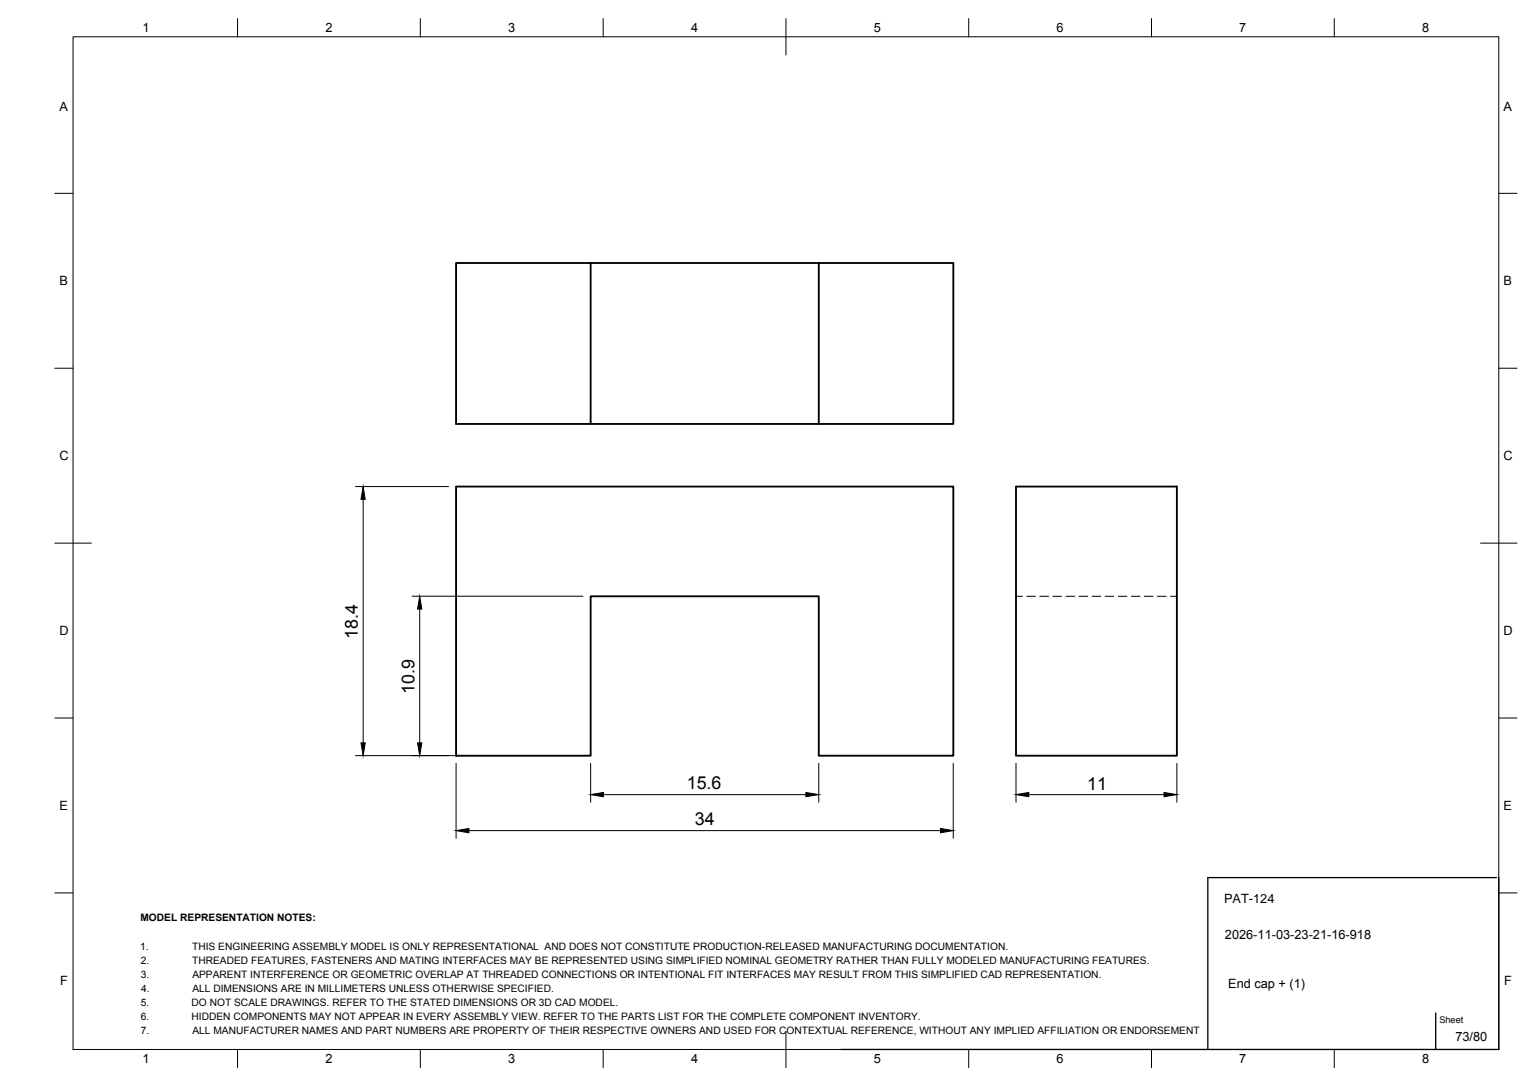
ISO-10303-21;
HEADER;
/* Generated by software containing ST-Developer
 * from STEP Tools, Inc. (www.steptools.com) 
 */

FILE_DESCRIPTION(
/* description */ ('XY cross-slide table'),
/* implementation_level */ '2;1');

FILE_NAME(
/* name */ 'End cap + (1).step',
/* time_stamp */ '2026-10-28T03:22:46-07:00',
/* author */ (''),
/* organization */ (''),
/* preprocessor_version */ 'ST-DEVELOPER v20.2',
/* originating_system */ 'Autodesk Translation Framework v15.17.0.0',
/* authorisation */ '');

FILE_SCHEMA (('AUTOMOTIVE_DESIGN { 1 0 10303 214 3 1 1 }'));
ENDSEC;

DATA;
#10=MECHANICAL_DESIGN_GEOMETRIC_PRESENTATION_REPRESENTATION('',(#1766),#62984);
#1570=SHAPE_REPRESENTATION_RELATIONSHIP('SRR','None',#63429,#1653);
#1653=ADVANCED_BREP_SHAPE_REPRESENTATION('',(#1874),#62966);
#1766=STYLED_ITEM('',(#63905),#1874);
#1874=MANIFOLD_SOLID_BREP('Body1',#23065);
#2749=PLANE('',#25946);
#2750=PLANE('',#25947);
#2751=PLANE('',#25948);
#2752=PLANE('',#25949);
#2753=PLANE('',#25950);
#2754=PLANE('',#25951);
#2755=PLANE('',#25952);
#2756=PLANE('',#25953);
#2757=PLANE('',#25954);
#2758=PLANE('',#25955);
#3857=FACE_OUTER_BOUND('',#5541,.T.);
#3858=FACE_OUTER_BOUND('',#5542,.T.);
#3859=FACE_OUTER_BOUND('',#5543,.T.);
#3860=FACE_OUTER_BOUND('',#5544,.T.);
#3861=FACE_OUTER_BOUND('',#5545,.T.);
#3862=FACE_OUTER_BOUND('',#5546,.T.);
#3863=FACE_OUTER_BOUND('',#5547,.T.);
#3864=FACE_OUTER_BOUND('',#5548,.T.);
#3865=FACE_OUTER_BOUND('',#5549,.T.);
#3866=FACE_OUTER_BOUND('',#5550,.T.);
#5541=EDGE_LOOP('',(#19434,#19435,#19436,#19437));
#5542=EDGE_LOOP('',(#19438,#19439,#19440,#19441));
#5543=EDGE_LOOP('',(#19442,#19443,#19444,#19445));
#5544=EDGE_LOOP('',(#19446,#19447,#19448,#19449));
#5545=EDGE_LOOP('',(#19450,#19451,#19452,#19453));
#5546=EDGE_LOOP('',(#19454,#19455,#19456,#19457));
#5547=EDGE_LOOP('',(#19458,#19459,#19460,#19461));
#5548=EDGE_LOOP('',(#19462,#19463,#19464,#19465));
#5549=EDGE_LOOP('',(#19466,#19467,#19468,#19469,#19470,#19471,#19472,#19473));
#5550=EDGE_LOOP('',(#19474,#19475,#19476,#19477,#19478,#19479,#19480,#19481));
#7004=LINE('',#50067,#8491);
#7005=LINE('',#50069,#8492);
#7006=LINE('',#50071,#8493);
#7007=LINE('',#50072,#8494);
#7008=LINE('',#50075,#8495);
#7009=LINE('',#50077,#8496);
#7010=LINE('',#50078,#8497);
#7011=LINE('',#50081,#8498);
#7012=LINE('',#50083,#8499);
#7013=LINE('',#50084,#8500);
#7014=LINE('',#50087,#8501);
#7015=LINE('',#50089,#8502);
#7016=LINE('',#50090,#8503);
#7017=LINE('',#50093,#8504);
#7018=LINE('',#50095,#8505);
#7019=LINE('',#50096,#8506);
#7020=LINE('',#50099,#8507);
#7021=LINE('',#50101,#8508);
#7022=LINE('',#50102,#8509);
#7023=LINE('',#50105,#8510);
#7024=LINE('',#50107,#8511);
#7025=LINE('',#50108,#8512);
#7026=LINE('',#50110,#8513);
#7027=LINE('',#50111,#8514);
#8491=VECTOR('',#31453,1.);
#8492=VECTOR('',#31454,1.);
#8493=VECTOR('',#31455,1.);
#8494=VECTOR('',#31456,1.);
#8495=VECTOR('',#31459,1.);
#8496=VECTOR('',#31460,1.);
#8497=VECTOR('',#31461,1.);
#8498=VECTOR('',#31464,1.);
#8499=VECTOR('',#31465,1.);
#8500=VECTOR('',#31466,1.);
#8501=VECTOR('',#31469,1.);
#8502=VECTOR('',#31470,1.);
#8503=VECTOR('',#31471,1.);
#8504=VECTOR('',#31474,1.);
#8505=VECTOR('',#31475,1.);
#8506=VECTOR('',#31476,1.);
#8507=VECTOR('',#31479,1.);
#8508=VECTOR('',#31480,1.);
#8509=VECTOR('',#31481,1.);
#8510=VECTOR('',#31484,1.);
#8511=VECTOR('',#31485,1.);
#8512=VECTOR('',#31486,1.);
#8513=VECTOR('',#31489,1.);
#8514=VECTOR('',#31490,1.);
#11306=VERTEX_POINT('',#50065);
#11307=VERTEX_POINT('',#50066);
#11308=VERTEX_POINT('',#50068);
#11309=VERTEX_POINT('',#50070);
#11310=VERTEX_POINT('',#50074);
#11311=VERTEX_POINT('',#50076);
#11312=VERTEX_POINT('',#50080);
#11313=VERTEX_POINT('',#50082);
#11314=VERTEX_POINT('',#50086);
#11315=VERTEX_POINT('',#50088);
#11316=VERTEX_POINT('',#50092);
#11317=VERTEX_POINT('',#50094);
#11318=VERTEX_POINT('',#50098);
#11319=VERTEX_POINT('',#50100);
#11320=VERTEX_POINT('',#50104);
#11321=VERTEX_POINT('',#50106);
#14101=EDGE_CURVE('',#11306,#11307,#7004,.T.);
#14102=EDGE_CURVE('',#11307,#11308,#7005,.T.);
#14103=EDGE_CURVE('',#11309,#11308,#7006,.T.);
#14104=EDGE_CURVE('',#11306,#11309,#7007,.T.);
#14105=EDGE_CURVE('',#11310,#11306,#7008,.T.);
#14106=EDGE_CURVE('',#11311,#11309,#7009,.T.);
#14107=EDGE_CURVE('',#11310,#11311,#7010,.T.);
#14108=EDGE_CURVE('',#11312,#11310,#7011,.T.);
#14109=EDGE_CURVE('',#11313,#11311,#7012,.T.);
#14110=EDGE_CURVE('',#11312,#11313,#7013,.T.);
#14111=EDGE_CURVE('',#11314,#11312,#7014,.T.);
#14112=EDGE_CURVE('',#11315,#11313,#7015,.T.);
#14113=EDGE_CURVE('',#11314,#11315,#7016,.T.);
#14114=EDGE_CURVE('',#11316,#11314,#7017,.T.);
#14115=EDGE_CURVE('',#11317,#11315,#7018,.T.);
#14116=EDGE_CURVE('',#11316,#11317,#7019,.T.);
#14117=EDGE_CURVE('',#11318,#11316,#7020,.T.);
#14118=EDGE_CURVE('',#11319,#11317,#7021,.T.);
#14119=EDGE_CURVE('',#11318,#11319,#7022,.T.);
#14120=EDGE_CURVE('',#11320,#11318,#7023,.T.);
#14121=EDGE_CURVE('',#11321,#11319,#7024,.T.);
#14122=EDGE_CURVE('',#11320,#11321,#7025,.T.);
#14123=EDGE_CURVE('',#11307,#11320,#7026,.T.);
#14124=EDGE_CURVE('',#11308,#11321,#7027,.T.);
#19434=ORIENTED_EDGE('',*,*,#14101,.T.);
#19435=ORIENTED_EDGE('',*,*,#14102,.T.);
#19436=ORIENTED_EDGE('',*,*,#14103,.F.);
#19437=ORIENTED_EDGE('',*,*,#14104,.F.);
#19438=ORIENTED_EDGE('',*,*,#14105,.T.);
#19439=ORIENTED_EDGE('',*,*,#14104,.T.);
#19440=ORIENTED_EDGE('',*,*,#14106,.F.);
#19441=ORIENTED_EDGE('',*,*,#14107,.F.);
#19442=ORIENTED_EDGE('',*,*,#14108,.T.);
#19443=ORIENTED_EDGE('',*,*,#14107,.T.);
#19444=ORIENTED_EDGE('',*,*,#14109,.F.);
#19445=ORIENTED_EDGE('',*,*,#14110,.F.);
#19446=ORIENTED_EDGE('',*,*,#14111,.T.);
#19447=ORIENTED_EDGE('',*,*,#14110,.T.);
#19448=ORIENTED_EDGE('',*,*,#14112,.F.);
#19449=ORIENTED_EDGE('',*,*,#14113,.F.);
#19450=ORIENTED_EDGE('',*,*,#14114,.T.);
#19451=ORIENTED_EDGE('',*,*,#14113,.T.);
#19452=ORIENTED_EDGE('',*,*,#14115,.F.);
#19453=ORIENTED_EDGE('',*,*,#14116,.F.);
#19454=ORIENTED_EDGE('',*,*,#14117,.T.);
#19455=ORIENTED_EDGE('',*,*,#14116,.T.);
#19456=ORIENTED_EDGE('',*,*,#14118,.F.);
#19457=ORIENTED_EDGE('',*,*,#14119,.F.);
#19458=ORIENTED_EDGE('',*,*,#14120,.T.);
#19459=ORIENTED_EDGE('',*,*,#14119,.T.);
#19460=ORIENTED_EDGE('',*,*,#14121,.F.);
#19461=ORIENTED_EDGE('',*,*,#14122,.F.);
#19462=ORIENTED_EDGE('',*,*,#14123,.T.);
#19463=ORIENTED_EDGE('',*,*,#14122,.T.);
#19464=ORIENTED_EDGE('',*,*,#14124,.F.);
#19465=ORIENTED_EDGE('',*,*,#14102,.F.);
#19466=ORIENTED_EDGE('',*,*,#14124,.T.);
#19467=ORIENTED_EDGE('',*,*,#14121,.T.);
#19468=ORIENTED_EDGE('',*,*,#14118,.T.);
#19469=ORIENTED_EDGE('',*,*,#14115,.T.);
#19470=ORIENTED_EDGE('',*,*,#14112,.T.);
#19471=ORIENTED_EDGE('',*,*,#14109,.T.);
#19472=ORIENTED_EDGE('',*,*,#14106,.T.);
#19473=ORIENTED_EDGE('',*,*,#14103,.T.);
#19474=ORIENTED_EDGE('',*,*,#14123,.F.);
#19475=ORIENTED_EDGE('',*,*,#14101,.F.);
#19476=ORIENTED_EDGE('',*,*,#14105,.F.);
#19477=ORIENTED_EDGE('',*,*,#14108,.F.);
#19478=ORIENTED_EDGE('',*,*,#14111,.F.);
#19479=ORIENTED_EDGE('',*,*,#14114,.F.);
#19480=ORIENTED_EDGE('',*,*,#14117,.F.);
#19481=ORIENTED_EDGE('',*,*,#14120,.F.);
#22638=ADVANCED_FACE('',(#3857),#2749,.T.);
#22639=ADVANCED_FACE('',(#3858),#2750,.T.);
#22640=ADVANCED_FACE('',(#3859),#2751,.T.);
#22641=ADVANCED_FACE('',(#3860),#2752,.T.);
#22642=ADVANCED_FACE('',(#3861),#2753,.T.);
#22643=ADVANCED_FACE('',(#3862),#2754,.T.);
#22644=ADVANCED_FACE('',(#3863),#2755,.T.);
#22645=ADVANCED_FACE('',(#3864),#2756,.T.);
#22646=ADVANCED_FACE('',(#3865),#2757,.T.);
#22647=ADVANCED_FACE('',(#3866),#2758,.F.);
#23065=CLOSED_SHELL('',(#22638,#22639,#22640,#22641,#22642,#22643,#22644,
#22645,#22646,#22647));
#25945=AXIS2_PLACEMENT_3D('',#50063,#31449,#31450);
#25946=AXIS2_PLACEMENT_3D('',#50064,#31451,#31452);
#25947=AXIS2_PLACEMENT_3D('',#50073,#31457,#31458);
#25948=AXIS2_PLACEMENT_3D('',#50079,#31462,#31463);
#25949=AXIS2_PLACEMENT_3D('',#50085,#31467,#31468);
#25950=AXIS2_PLACEMENT_3D('',#50091,#31472,#31473);
#25951=AXIS2_PLACEMENT_3D('',#50097,#31477,#31478);
#25952=AXIS2_PLACEMENT_3D('',#50103,#31482,#31483);
#25953=AXIS2_PLACEMENT_3D('',#50109,#31487,#31488);
#25954=AXIS2_PLACEMENT_3D('',#50112,#31491,#31492);
#25955=AXIS2_PLACEMENT_3D('',#50113,#31493,#31494);
#31449=DIRECTION('axis',(0.,0.,1.));
#31450=DIRECTION('refdir',(1.,0.,0.));
#31451=DIRECTION('center_axis',(0.,0.,1.));
#31452=DIRECTION('ref_axis',(0.,-1.,0.));
#31453=DIRECTION('',(0.,-1.,0.));
#31454=DIRECTION('',(1.,0.,0.));
#31455=DIRECTION('',(0.,-1.,0.));
#31456=DIRECTION('',(1.,0.,0.));
#31457=DIRECTION('center_axis',(0.,1.,0.));
#31458=DIRECTION('ref_axis',(0.,0.,1.));
#31459=DIRECTION('',(0.,0.,1.));
#31460=DIRECTION('',(0.,0.,1.));
#31461=DIRECTION('',(1.,0.,0.));
#31462=DIRECTION('center_axis',(0.,0.,-1.));
#31463=DIRECTION('ref_axis',(0.,1.,0.));
#31464=DIRECTION('',(0.,1.,0.));
#31465=DIRECTION('',(0.,1.,0.));
#31466=DIRECTION('',(1.,0.,0.));
#31467=DIRECTION('center_axis',(0.,-1.,0.));
#31468=DIRECTION('ref_axis',(0.,0.,-1.));
#31469=DIRECTION('',(0.,0.,-1.));
#31470=DIRECTION('',(0.,0.,-1.));
#31471=DIRECTION('',(1.,0.,0.));
#31472=DIRECTION('center_axis',(0.,0.,-1.));
#31473=DIRECTION('ref_axis',(0.,1.,0.));
#31474=DIRECTION('',(0.,1.,0.));
#31475=DIRECTION('',(0.,1.,0.));
#31476=DIRECTION('',(1.,0.,0.));
#31477=DIRECTION('center_axis',(0.,1.,0.));
#31478=DIRECTION('ref_axis',(0.,0.,1.));
#31479=DIRECTION('',(0.,0.,1.));
#31480=DIRECTION('',(0.,0.,1.));
#31481=DIRECTION('',(1.,0.,0.));
#31482=DIRECTION('center_axis',(0.,0.,-1.));
#31483=DIRECTION('ref_axis',(0.,1.,0.));
#31484=DIRECTION('',(0.,1.,0.));
#31485=DIRECTION('',(0.,1.,0.));
#31486=DIRECTION('',(1.,0.,0.));
#31487=DIRECTION('center_axis',(0.,-1.,0.));
#31488=DIRECTION('ref_axis',(0.,0.,-1.));
#31489=DIRECTION('',(0.,0.,-1.));
#31490=DIRECTION('',(0.,0.,-1.));
#31491=DIRECTION('center_axis',(1.,0.,0.));
#31492=DIRECTION('ref_axis',(0.,0.,-1.));
#31493=DIRECTION('center_axis',(1.,0.,0.));
#31494=DIRECTION('ref_axis',(0.,0.,-1.));
#50063=CARTESIAN_POINT('',(0.,0.,0.));
#50064=CARTESIAN_POINT('Origin',(1.97,1.7,2.3));
#50065=CARTESIAN_POINT('',(1.97,1.7,2.3));
#50066=CARTESIAN_POINT('',(1.97,-1.7,2.3));
#50067=CARTESIAN_POINT('',(1.97,1.7,2.3));
#50068=CARTESIAN_POINT('',(3.07,-1.7,2.3));
#50069=CARTESIAN_POINT('',(1.97,-1.7,2.3));
#50070=CARTESIAN_POINT('',(3.07,1.7,2.3));
#50071=CARTESIAN_POINT('',(3.07,1.7,2.3));
#50072=CARTESIAN_POINT('',(1.97,1.7,2.3));
#50073=CARTESIAN_POINT('Origin',(1.97,1.7,0.46));
#50074=CARTESIAN_POINT('',(1.97,1.7,0.46));
#50075=CARTESIAN_POINT('',(1.97,1.7,0.46));
#50076=CARTESIAN_POINT('',(3.07,1.7,0.46));
#50077=CARTESIAN_POINT('',(3.07,1.7,0.46));
#50078=CARTESIAN_POINT('',(1.97,1.7,0.46));
#50079=CARTESIAN_POINT('Origin',(1.97,0.78,0.46));
#50080=CARTESIAN_POINT('',(1.97,0.78,0.46));
#50081=CARTESIAN_POINT('',(1.97,0.78,0.46));
#50082=CARTESIAN_POINT('',(3.07,0.78,0.46));
#50083=CARTESIAN_POINT('',(3.07,0.78,0.46));
#50084=CARTESIAN_POINT('',(1.97,0.78,0.46));
#50085=CARTESIAN_POINT('Origin',(1.97,0.78,1.55));
#50086=CARTESIAN_POINT('',(1.97,0.78,1.55));
#50087=CARTESIAN_POINT('',(1.97,0.78,1.55));
#50088=CARTESIAN_POINT('',(3.07,0.78,1.55));
#50089=CARTESIAN_POINT('',(3.07,0.78,1.55));
#50090=CARTESIAN_POINT('',(1.97,0.78,1.55));
#50091=CARTESIAN_POINT('Origin',(1.97,-0.78,1.55));
#50092=CARTESIAN_POINT('',(1.97,-0.78,1.55));
#50093=CARTESIAN_POINT('',(1.97,-0.78,1.55));
#50094=CARTESIAN_POINT('',(3.07,-0.78,1.55));
#50095=CARTESIAN_POINT('',(3.07,-0.78,1.55));
#50096=CARTESIAN_POINT('',(1.97,-0.78,1.55));
#50097=CARTESIAN_POINT('Origin',(1.97,-0.78,0.46));
#50098=CARTESIAN_POINT('',(1.97,-0.78,0.46));
#50099=CARTESIAN_POINT('',(1.97,-0.78,0.46));
#50100=CARTESIAN_POINT('',(3.07,-0.78,0.46));
#50101=CARTESIAN_POINT('',(3.07,-0.78,0.46));
#50102=CARTESIAN_POINT('',(1.97,-0.78,0.46));
#50103=CARTESIAN_POINT('Origin',(1.97,-1.7,0.46));
#50104=CARTESIAN_POINT('',(1.97,-1.7,0.46));
#50105=CARTESIAN_POINT('',(1.97,-1.7,0.46));
#50106=CARTESIAN_POINT('',(3.07,-1.7,0.46));
#50107=CARTESIAN_POINT('',(3.07,-1.7,0.46));
#50108=CARTESIAN_POINT('',(1.97,-1.7,0.46));
#50109=CARTESIAN_POINT('Origin',(1.97,-1.7,2.3));
#50110=CARTESIAN_POINT('',(1.97,-1.7,2.3));
#50111=CARTESIAN_POINT('',(3.07,-1.7,2.3));
#50112=CARTESIAN_POINT('Origin',(3.07,0.,1.38));
#50113=CARTESIAN_POINT('Origin',(1.97,0.,1.38));
#62867=UNCERTAINTY_MEASURE_WITH_UNIT(LENGTH_MEASURE(0.001),#62985,
'DISTANCE_ACCURACY_VALUE',
'Maximum model space distance between geometric entities at asserted c
onnectivities');
#62885=UNCERTAINTY_MEASURE_WITH_UNIT(LENGTH_MEASURE(0.001),#62985,
'DISTANCE_ACCURACY_VALUE',
'Maximum model space distance between geometric entities at asserted c
onnectivities');
#62966=(
GEOMETRIC_REPRESENTATION_CONTEXT(3)
GLOBAL_UNCERTAINTY_ASSIGNED_CONTEXT((#62867))
GLOBAL_UNIT_ASSIGNED_CONTEXT((#62985,#62987,#62988))
REPRESENTATION_CONTEXT('','3D')
);
#62984=(
GEOMETRIC_REPRESENTATION_CONTEXT(3)
GLOBAL_UNCERTAINTY_ASSIGNED_CONTEXT((#62885))
GLOBAL_UNIT_ASSIGNED_CONTEXT((#62985,#62987,#62988))
REPRESENTATION_CONTEXT('','3D')
);
#62985=(
LENGTH_UNIT()
NAMED_UNIT(*)
SI_UNIT(.CENTI.,.METRE.)
);
#62987=(
NAMED_UNIT(*)
PLANE_ANGLE_UNIT()
SI_UNIT($,.RADIAN.)
);
#62988=(
NAMED_UNIT(*)
SI_UNIT($,.STERADIAN.)
SOLID_ANGLE_UNIT()
);
#63069=SHAPE_DEFINITION_REPRESENTATION(#63257,#63429);
#63257=PRODUCT_DEFINITION_SHAPE('',$,#63528);
#63429=SHAPE_REPRESENTATION('',(#25945),#62966);
#63447=PRODUCT_DEFINITION_CONTEXT('part definition',#63743,'design');
#63528=PRODUCT_DEFINITION('End cap + (1)','End cap + (1)',#63626,#63447);
#63626=PRODUCT_DEFINITION_FORMATION('',$,#63825);
#63743=APPLICATION_CONTEXT(
'Core Data for Automotive Mechanical Design Process');
#63744=PRODUCT_CONTEXT('part definition',#63743,'mechanical');
#63825=PRODUCT('End cap + (1)','End cap + (1)','End cap + (1)',(#63744));
#63899=COLOUR_RGB('Sky Blue',0.24,0.69,0.87);
#63900=FILL_AREA_STYLE_COLOUR('',#63899);
#63901=FILL_AREA_STYLE('',(#63900));
#63902=SURFACE_STYLE_FILL_AREA(#63901);
#63903=SURFACE_SIDE_STYLE('',(#63902));
#63904=SURFACE_STYLE_USAGE(.BOTH.,#63903);
#63905=PRESENTATION_STYLE_ASSIGNMENT((#63904));
ENDSEC;
END-ISO-10303-21;
